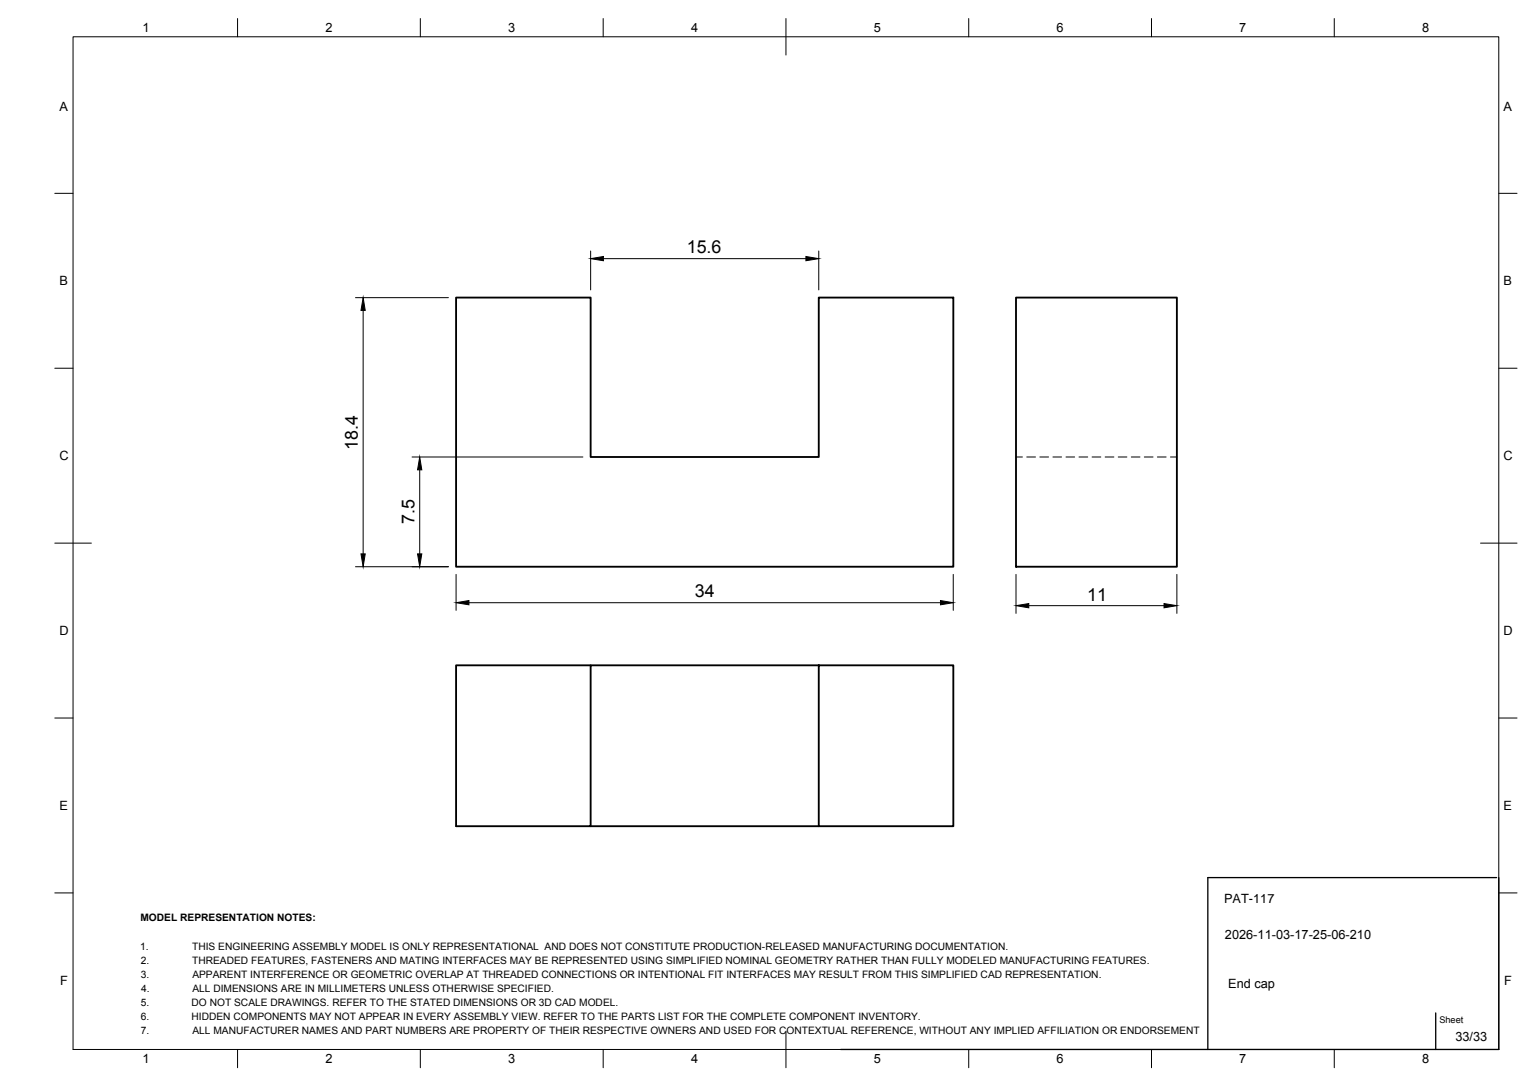
ISO-10303-21;
HEADER;
/* Generated by software containing ST-Developer
 * from STEP Tools, Inc. (www.steptools.com) 
 */

FILE_DESCRIPTION(
/* description */ ('Counterbalanced vertical column'),
/* implementation_level */ '2;1');

FILE_NAME(
/* name */ 'End cap.step',
/* time_stamp */ '2026-10-29T16:47:22-07:00',
/* author */ (''),
/* organization */ (''),
/* preprocessor_version */ 'ST-DEVELOPER v20.2',
/* originating_system */ 'Autodesk Translation Framework v15.17.0.0',
/* authorisation */ '');

FILE_SCHEMA (('AUTOMOTIVE_DESIGN { 1 0 10303 214 3 1 1 }'));
ENDSEC;

DATA;
#10=MECHANICAL_DESIGN_GEOMETRIC_PRESENTATION_REPRESENTATION('',(#382),#15040);
#312=SHAPE_REPRESENTATION_RELATIONSHIP('SRR','None',#15218,#347);
#347=ADVANCED_BREP_SHAPE_REPRESENTATION('',(#415),#15037);
#382=STYLED_ITEM('',(#15471),#415);
#415=MANIFOLD_SOLID_BREP('Body1',#7107);
#794=PLANE('',#8102);
#795=PLANE('',#8103);
#796=PLANE('',#8104);
#797=PLANE('',#8105);
#798=PLANE('',#8106);
#799=PLANE('',#8107);
#800=PLANE('',#8108);
#801=PLANE('',#8109);
#802=PLANE('',#8110);
#803=PLANE('',#8111);
#1188=FACE_OUTER_BOUND('',#1706,.T.);
#1189=FACE_OUTER_BOUND('',#1707,.T.);
#1190=FACE_OUTER_BOUND('',#1708,.T.);
#1191=FACE_OUTER_BOUND('',#1709,.T.);
#1192=FACE_OUTER_BOUND('',#1710,.T.);
#1193=FACE_OUTER_BOUND('',#1711,.T.);
#1194=FACE_OUTER_BOUND('',#1712,.T.);
#1195=FACE_OUTER_BOUND('',#1713,.T.);
#1196=FACE_OUTER_BOUND('',#1714,.T.);
#1197=FACE_OUTER_BOUND('',#1715,.T.);
#1706=EDGE_LOOP('',(#6402,#6403,#6404,#6405));
#1707=EDGE_LOOP('',(#6406,#6407,#6408,#6409));
#1708=EDGE_LOOP('',(#6410,#6411,#6412,#6413));
#1709=EDGE_LOOP('',(#6414,#6415,#6416,#6417));
#1710=EDGE_LOOP('',(#6418,#6419,#6420,#6421));
#1711=EDGE_LOOP('',(#6422,#6423,#6424,#6425));
#1712=EDGE_LOOP('',(#6426,#6427,#6428,#6429));
#1713=EDGE_LOOP('',(#6430,#6431,#6432,#6433));
#1714=EDGE_LOOP('',(#6434,#6435,#6436,#6437,#6438,#6439,#6440,#6441));
#1715=EDGE_LOOP('',(#6442,#6443,#6444,#6445,#6446,#6447,#6448,#6449));
#2351=LINE('',#14719,#3022);
#2352=LINE('',#14721,#3023);
#2353=LINE('',#14723,#3024);
#2354=LINE('',#14724,#3025);
#2355=LINE('',#14727,#3026);
#2356=LINE('',#14729,#3027);
#2357=LINE('',#14730,#3028);
#2358=LINE('',#14733,#3029);
#2359=LINE('',#14735,#3030);
#2360=LINE('',#14736,#3031);
#2361=LINE('',#14739,#3032);
#2362=LINE('',#14741,#3033);
#2363=LINE('',#14742,#3034);
#2364=LINE('',#14745,#3035);
#2365=LINE('',#14747,#3036);
#2366=LINE('',#14748,#3037);
#2367=LINE('',#14751,#3038);
#2368=LINE('',#14753,#3039);
#2369=LINE('',#14754,#3040);
#2370=LINE('',#14757,#3041);
#2371=LINE('',#14759,#3042);
#2372=LINE('',#14760,#3043);
#2373=LINE('',#14762,#3044);
#2374=LINE('',#14763,#3045);
#3022=VECTOR('',#10031,1.);
#3023=VECTOR('',#10032,1.);
#3024=VECTOR('',#10033,1.);
#3025=VECTOR('',#10034,1.);
#3026=VECTOR('',#10037,1.);
#3027=VECTOR('',#10038,1.);
#3028=VECTOR('',#10039,1.);
#3029=VECTOR('',#10042,1.);
#3030=VECTOR('',#10043,1.);
#3031=VECTOR('',#10044,1.);
#3032=VECTOR('',#10047,1.);
#3033=VECTOR('',#10048,1.);
#3034=VECTOR('',#10049,1.);
#3035=VECTOR('',#10052,1.);
#3036=VECTOR('',#10053,1.);
#3037=VECTOR('',#10054,1.);
#3038=VECTOR('',#10057,1.);
#3039=VECTOR('',#10058,1.);
#3040=VECTOR('',#10059,1.);
#3041=VECTOR('',#10062,1.);
#3042=VECTOR('',#10063,1.);
#3043=VECTOR('',#10064,1.);
#3044=VECTOR('',#10067,1.);
#3045=VECTOR('',#10068,1.);
#3840=VERTEX_POINT('',#14717);
#3841=VERTEX_POINT('',#14718);
#3842=VERTEX_POINT('',#14720);
#3843=VERTEX_POINT('',#14722);
#3844=VERTEX_POINT('',#14726);
#3845=VERTEX_POINT('',#14728);
#3846=VERTEX_POINT('',#14732);
#3847=VERTEX_POINT('',#14734);
#3848=VERTEX_POINT('',#14738);
#3849=VERTEX_POINT('',#14740);
#3850=VERTEX_POINT('',#14744);
#3851=VERTEX_POINT('',#14746);
#3852=VERTEX_POINT('',#14750);
#3853=VERTEX_POINT('',#14752);
#3854=VERTEX_POINT('',#14756);
#3855=VERTEX_POINT('',#14758);
#4702=EDGE_CURVE('',#3840,#3841,#2351,.T.);
#4703=EDGE_CURVE('',#3840,#3842,#2352,.T.);
#4704=EDGE_CURVE('',#3843,#3842,#2353,.T.);
#4705=EDGE_CURVE('',#3841,#3843,#2354,.T.);
#4706=EDGE_CURVE('',#3841,#3844,#2355,.T.);
#4707=EDGE_CURVE('',#3845,#3843,#2356,.T.);
#4708=EDGE_CURVE('',#3844,#3845,#2357,.T.);
#4709=EDGE_CURVE('',#3844,#3846,#2358,.T.);
#4710=EDGE_CURVE('',#3847,#3845,#2359,.T.);
#4711=EDGE_CURVE('',#3846,#3847,#2360,.T.);
#4712=EDGE_CURVE('',#3846,#3848,#2361,.T.);
#4713=EDGE_CURVE('',#3849,#3847,#2362,.T.);
#4714=EDGE_CURVE('',#3848,#3849,#2363,.T.);
#4715=EDGE_CURVE('',#3848,#3850,#2364,.T.);
#4716=EDGE_CURVE('',#3851,#3849,#2365,.T.);
#4717=EDGE_CURVE('',#3850,#3851,#2366,.T.);
#4718=EDGE_CURVE('',#3850,#3852,#2367,.T.);
#4719=EDGE_CURVE('',#3853,#3851,#2368,.T.);
#4720=EDGE_CURVE('',#3852,#3853,#2369,.T.);
#4721=EDGE_CURVE('',#3852,#3854,#2370,.T.);
#4722=EDGE_CURVE('',#3855,#3853,#2371,.T.);
#4723=EDGE_CURVE('',#3854,#3855,#2372,.T.);
#4724=EDGE_CURVE('',#3854,#3840,#2373,.T.);
#4725=EDGE_CURVE('',#3842,#3855,#2374,.T.);
#6402=ORIENTED_EDGE('',*,*,#4702,.F.);
#6403=ORIENTED_EDGE('',*,*,#4703,.T.);
#6404=ORIENTED_EDGE('',*,*,#4704,.F.);
#6405=ORIENTED_EDGE('',*,*,#4705,.F.);
#6406=ORIENTED_EDGE('',*,*,#4706,.F.);
#6407=ORIENTED_EDGE('',*,*,#4705,.T.);
#6408=ORIENTED_EDGE('',*,*,#4707,.F.);
#6409=ORIENTED_EDGE('',*,*,#4708,.F.);
#6410=ORIENTED_EDGE('',*,*,#4709,.F.);
#6411=ORIENTED_EDGE('',*,*,#4708,.T.);
#6412=ORIENTED_EDGE('',*,*,#4710,.F.);
#6413=ORIENTED_EDGE('',*,*,#4711,.F.);
#6414=ORIENTED_EDGE('',*,*,#4712,.F.);
#6415=ORIENTED_EDGE('',*,*,#4711,.T.);
#6416=ORIENTED_EDGE('',*,*,#4713,.F.);
#6417=ORIENTED_EDGE('',*,*,#4714,.F.);
#6418=ORIENTED_EDGE('',*,*,#4715,.F.);
#6419=ORIENTED_EDGE('',*,*,#4714,.T.);
#6420=ORIENTED_EDGE('',*,*,#4716,.F.);
#6421=ORIENTED_EDGE('',*,*,#4717,.F.);
#6422=ORIENTED_EDGE('',*,*,#4718,.F.);
#6423=ORIENTED_EDGE('',*,*,#4717,.T.);
#6424=ORIENTED_EDGE('',*,*,#4719,.F.);
#6425=ORIENTED_EDGE('',*,*,#4720,.F.);
#6426=ORIENTED_EDGE('',*,*,#4721,.F.);
#6427=ORIENTED_EDGE('',*,*,#4720,.T.);
#6428=ORIENTED_EDGE('',*,*,#4722,.F.);
#6429=ORIENTED_EDGE('',*,*,#4723,.F.);
#6430=ORIENTED_EDGE('',*,*,#4724,.F.);
#6431=ORIENTED_EDGE('',*,*,#4723,.T.);
#6432=ORIENTED_EDGE('',*,*,#4725,.F.);
#6433=ORIENTED_EDGE('',*,*,#4703,.F.);
#6434=ORIENTED_EDGE('',*,*,#4724,.T.);
#6435=ORIENTED_EDGE('',*,*,#4702,.T.);
#6436=ORIENTED_EDGE('',*,*,#4706,.T.);
#6437=ORIENTED_EDGE('',*,*,#4709,.T.);
#6438=ORIENTED_EDGE('',*,*,#4712,.T.);
#6439=ORIENTED_EDGE('',*,*,#4715,.T.);
#6440=ORIENTED_EDGE('',*,*,#4718,.T.);
#6441=ORIENTED_EDGE('',*,*,#4721,.T.);
#6442=ORIENTED_EDGE('',*,*,#4725,.T.);
#6443=ORIENTED_EDGE('',*,*,#4722,.T.);
#6444=ORIENTED_EDGE('',*,*,#4719,.T.);
#6445=ORIENTED_EDGE('',*,*,#4716,.T.);
#6446=ORIENTED_EDGE('',*,*,#4713,.T.);
#6447=ORIENTED_EDGE('',*,*,#4710,.T.);
#6448=ORIENTED_EDGE('',*,*,#4707,.T.);
#6449=ORIENTED_EDGE('',*,*,#4704,.T.);
#7030=ADVANCED_FACE('',(#1188),#794,.T.);
#7031=ADVANCED_FACE('',(#1189),#795,.T.);
#7032=ADVANCED_FACE('',(#1190),#796,.T.);
#7033=ADVANCED_FACE('',(#1191),#797,.T.);
#7034=ADVANCED_FACE('',(#1192),#798,.T.);
#7035=ADVANCED_FACE('',(#1193),#799,.T.);
#7036=ADVANCED_FACE('',(#1194),#800,.T.);
#7037=ADVANCED_FACE('',(#1195),#801,.T.);
#7038=ADVANCED_FACE('',(#1196),#802,.T.);
#7039=ADVANCED_FACE('',(#1197),#803,.T.);
#7107=CLOSED_SHELL('',(#7030,#7031,#7032,#7033,#7034,#7035,#7036,#7037,
#7038,#7039));
#8101=AXIS2_PLACEMENT_3D('',#14715,#10027,#10028);
#8102=AXIS2_PLACEMENT_3D('',#14716,#10029,#10030);
#8103=AXIS2_PLACEMENT_3D('',#14725,#10035,#10036);
#8104=AXIS2_PLACEMENT_3D('',#14731,#10040,#10041);
#8105=AXIS2_PLACEMENT_3D('',#14737,#10045,#10046);
#8106=AXIS2_PLACEMENT_3D('',#14743,#10050,#10051);
#8107=AXIS2_PLACEMENT_3D('',#14749,#10055,#10056);
#8108=AXIS2_PLACEMENT_3D('',#14755,#10060,#10061);
#8109=AXIS2_PLACEMENT_3D('',#14761,#10065,#10066);
#8110=AXIS2_PLACEMENT_3D('',#14764,#10069,#10070);
#8111=AXIS2_PLACEMENT_3D('',#14765,#10071,#10072);
#10027=DIRECTION('axis',(0.,0.,1.));
#10028=DIRECTION('refdir',(1.,0.,0.));
#10029=DIRECTION('center_axis',(0.,0.,-1.));
#10030=DIRECTION('ref_axis',(0.,-1.,0.));
#10031=DIRECTION('',(0.,1.,0.));
#10032=DIRECTION('',(-1.,0.,0.));
#10033=DIRECTION('',(0.,-1.,0.));
#10034=DIRECTION('',(-1.,0.,0.));
#10035=DIRECTION('center_axis',(0.,1.,0.));
#10036=DIRECTION('ref_axis',(0.,0.,-1.));
#10037=DIRECTION('',(0.,0.,1.));
#10038=DIRECTION('',(0.,0.,-1.));
#10039=DIRECTION('',(-1.,0.,0.));
#10040=DIRECTION('center_axis',(0.,0.,-1.));
#10041=DIRECTION('ref_axis',(0.,-1.,0.));
#10042=DIRECTION('',(0.,1.,0.));
#10043=DIRECTION('',(0.,-1.,0.));
#10044=DIRECTION('',(-1.,0.,0.));
#10045=DIRECTION('center_axis',(0.,-1.,0.));
#10046=DIRECTION('ref_axis',(0.,0.,1.));
#10047=DIRECTION('',(0.,0.,-1.));
#10048=DIRECTION('',(0.,0.,1.));
#10049=DIRECTION('',(-1.,0.,0.));
#10050=DIRECTION('center_axis',(0.,0.,-1.));
#10051=DIRECTION('ref_axis',(0.,-1.,0.));
#10052=DIRECTION('',(0.,1.,0.));
#10053=DIRECTION('',(0.,-1.,0.));
#10054=DIRECTION('',(-1.,0.,0.));
#10055=DIRECTION('center_axis',(0.,1.,0.));
#10056=DIRECTION('ref_axis',(0.,0.,-1.));
#10057=DIRECTION('',(0.,0.,1.));
#10058=DIRECTION('',(0.,0.,-1.));
#10059=DIRECTION('',(-1.,0.,0.));
#10060=DIRECTION('center_axis',(0.,0.,1.));
#10061=DIRECTION('ref_axis',(0.,1.,0.));
#10062=DIRECTION('',(0.,-1.,0.));
#10063=DIRECTION('',(0.,1.,0.));
#10064=DIRECTION('',(-1.,0.,0.));
#10065=DIRECTION('center_axis',(0.,-1.,0.));
#10066=DIRECTION('ref_axis',(0.,0.,1.));
#10067=DIRECTION('',(0.,0.,-1.));
#10068=DIRECTION('',(0.,0.,1.));
#10069=DIRECTION('center_axis',(1.,0.,0.));
#10070=DIRECTION('ref_axis',(0.,0.,-1.));
#10071=DIRECTION('center_axis',(-1.,0.,0.));
#10072=DIRECTION('ref_axis',(0.,0.,1.));
#14715=CARTESIAN_POINT('',(0.,0.,0.));
#14716=CARTESIAN_POINT('Origin',(-1.97,-0.78,0.46));
#14717=CARTESIAN_POINT('',(-1.97,-1.7,0.46));
#14718=CARTESIAN_POINT('',(-1.97,-0.78,0.46));
#14719=CARTESIAN_POINT('',(-1.97,-1.7,0.46));
#14720=CARTESIAN_POINT('',(-3.07,-1.7,0.46));
#14721=CARTESIAN_POINT('',(-1.97,-1.7,0.46));
#14722=CARTESIAN_POINT('',(-3.07,-0.78,0.46));
#14723=CARTESIAN_POINT('',(-3.07,-1.7,0.46));
#14724=CARTESIAN_POINT('',(-1.97,-0.78,0.46));
#14725=CARTESIAN_POINT('Origin',(-1.97,-0.78,1.55));
#14726=CARTESIAN_POINT('',(-1.97,-0.78,1.55));
#14727=CARTESIAN_POINT('',(-1.97,-0.78,0.46));
#14728=CARTESIAN_POINT('',(-3.07,-0.78,1.55));
#14729=CARTESIAN_POINT('',(-3.07,-0.78,0.46));
#14730=CARTESIAN_POINT('',(-1.97,-0.78,1.55));
#14731=CARTESIAN_POINT('Origin',(-1.97,0.78,1.55));
#14732=CARTESIAN_POINT('',(-1.97,0.78,1.55));
#14733=CARTESIAN_POINT('',(-1.97,-0.78,1.55));
#14734=CARTESIAN_POINT('',(-3.07,0.78,1.55));
#14735=CARTESIAN_POINT('',(-3.07,-0.78,1.55));
#14736=CARTESIAN_POINT('',(-1.97,0.78,1.55));
#14737=CARTESIAN_POINT('Origin',(-1.97,0.78,0.46));
#14738=CARTESIAN_POINT('',(-1.97,0.78,0.46));
#14739=CARTESIAN_POINT('',(-1.97,0.78,1.55));
#14740=CARTESIAN_POINT('',(-3.07,0.78,0.46));
#14741=CARTESIAN_POINT('',(-3.07,0.78,1.55));
#14742=CARTESIAN_POINT('',(-1.97,0.78,0.46));
#14743=CARTESIAN_POINT('Origin',(-1.97,1.7,0.46));
#14744=CARTESIAN_POINT('',(-1.97,1.7,0.46));
#14745=CARTESIAN_POINT('',(-1.97,0.78,0.46));
#14746=CARTESIAN_POINT('',(-3.07,1.7,0.46));
#14747=CARTESIAN_POINT('',(-3.07,0.78,0.46));
#14748=CARTESIAN_POINT('',(-1.97,1.7,0.46));
#14749=CARTESIAN_POINT('Origin',(-1.97,1.7,2.3));
#14750=CARTESIAN_POINT('',(-1.97,1.7,2.3));
#14751=CARTESIAN_POINT('',(-1.97,1.7,0.46));
#14752=CARTESIAN_POINT('',(-3.07,1.7,2.3));
#14753=CARTESIAN_POINT('',(-3.07,1.7,0.46));
#14754=CARTESIAN_POINT('',(-1.97,1.7,2.3));
#14755=CARTESIAN_POINT('Origin',(-1.97,-1.7,2.3));
#14756=CARTESIAN_POINT('',(-1.97,-1.7,2.3));
#14757=CARTESIAN_POINT('',(-1.97,1.7,2.3));
#14758=CARTESIAN_POINT('',(-3.07,-1.7,2.3));
#14759=CARTESIAN_POINT('',(-3.07,1.7,2.3));
#14760=CARTESIAN_POINT('',(-1.97,-1.7,2.3));
#14761=CARTESIAN_POINT('Origin',(-1.97,-1.7,0.46));
#14762=CARTESIAN_POINT('',(-1.97,-1.7,2.3));
#14763=CARTESIAN_POINT('',(-3.07,-1.7,2.3));
#14764=CARTESIAN_POINT('Origin',(-1.97,0.,1.38));
#14765=CARTESIAN_POINT('Origin',(-3.07,0.,1.38));
#14997=UNCERTAINTY_MEASURE_WITH_UNIT(LENGTH_MEASURE(0.001),#15041,
'DISTANCE_ACCURACY_VALUE',
'Maximum model space distance between geometric entities at asserted c
onnectivities');
#15000=UNCERTAINTY_MEASURE_WITH_UNIT(LENGTH_MEASURE(0.001),#15041,
'DISTANCE_ACCURACY_VALUE',
'Maximum model space distance between geometric entities at asserted c
onnectivities');
#15037=(
GEOMETRIC_REPRESENTATION_CONTEXT(3)
GLOBAL_UNCERTAINTY_ASSIGNED_CONTEXT((#14997))
GLOBAL_UNIT_ASSIGNED_CONTEXT((#15041,#15043,#15044))
REPRESENTATION_CONTEXT('','3D')
);
#15040=(
GEOMETRIC_REPRESENTATION_CONTEXT(3)
GLOBAL_UNCERTAINTY_ASSIGNED_CONTEXT((#15000))
GLOBAL_UNIT_ASSIGNED_CONTEXT((#15041,#15043,#15044))
REPRESENTATION_CONTEXT('','3D')
);
#15041=(
LENGTH_UNIT()
NAMED_UNIT(*)
SI_UNIT(.CENTI.,.METRE.)
);
#15043=(
NAMED_UNIT(*)
PLANE_ANGLE_UNIT()
SI_UNIT($,.RADIAN.)
);
#15044=(
NAMED_UNIT(*)
SI_UNIT($,.STERADIAN.)
SOLID_ANGLE_UNIT()
);
#15081=SHAPE_DEFINITION_REPRESENTATION(#15120,#15218);
#15120=PRODUCT_DEFINITION_SHAPE('',$,#15258);
#15218=SHAPE_REPRESENTATION('',(#8101),#15037);
#15221=PRODUCT_DEFINITION_CONTEXT('part definition',#15340,'design');
#15258=PRODUCT_DEFINITION('End cap','End cap',#15297,#15221);
#15297=PRODUCT_DEFINITION_FORMATION('',$,#15378);
#15340=APPLICATION_CONTEXT(
'Core Data for Automotive Mechanical Design Process');
#15341=PRODUCT_CONTEXT('part definition',#15340,'mechanical');
#15378=PRODUCT('End cap','End cap','End cap',(#15341));
#15465=COLOUR_RGB('Off White',0.89,0.88,0.83);
#15466=FILL_AREA_STYLE_COLOUR('',#15465);
#15467=FILL_AREA_STYLE('',(#15466));
#15468=SURFACE_STYLE_FILL_AREA(#15467);
#15469=SURFACE_SIDE_STYLE('',(#15468));
#15470=SURFACE_STYLE_USAGE(.BOTH.,#15469);
#15471=PRESENTATION_STYLE_ASSIGNMENT((#15470));
ENDSEC;
END-ISO-10303-21;
